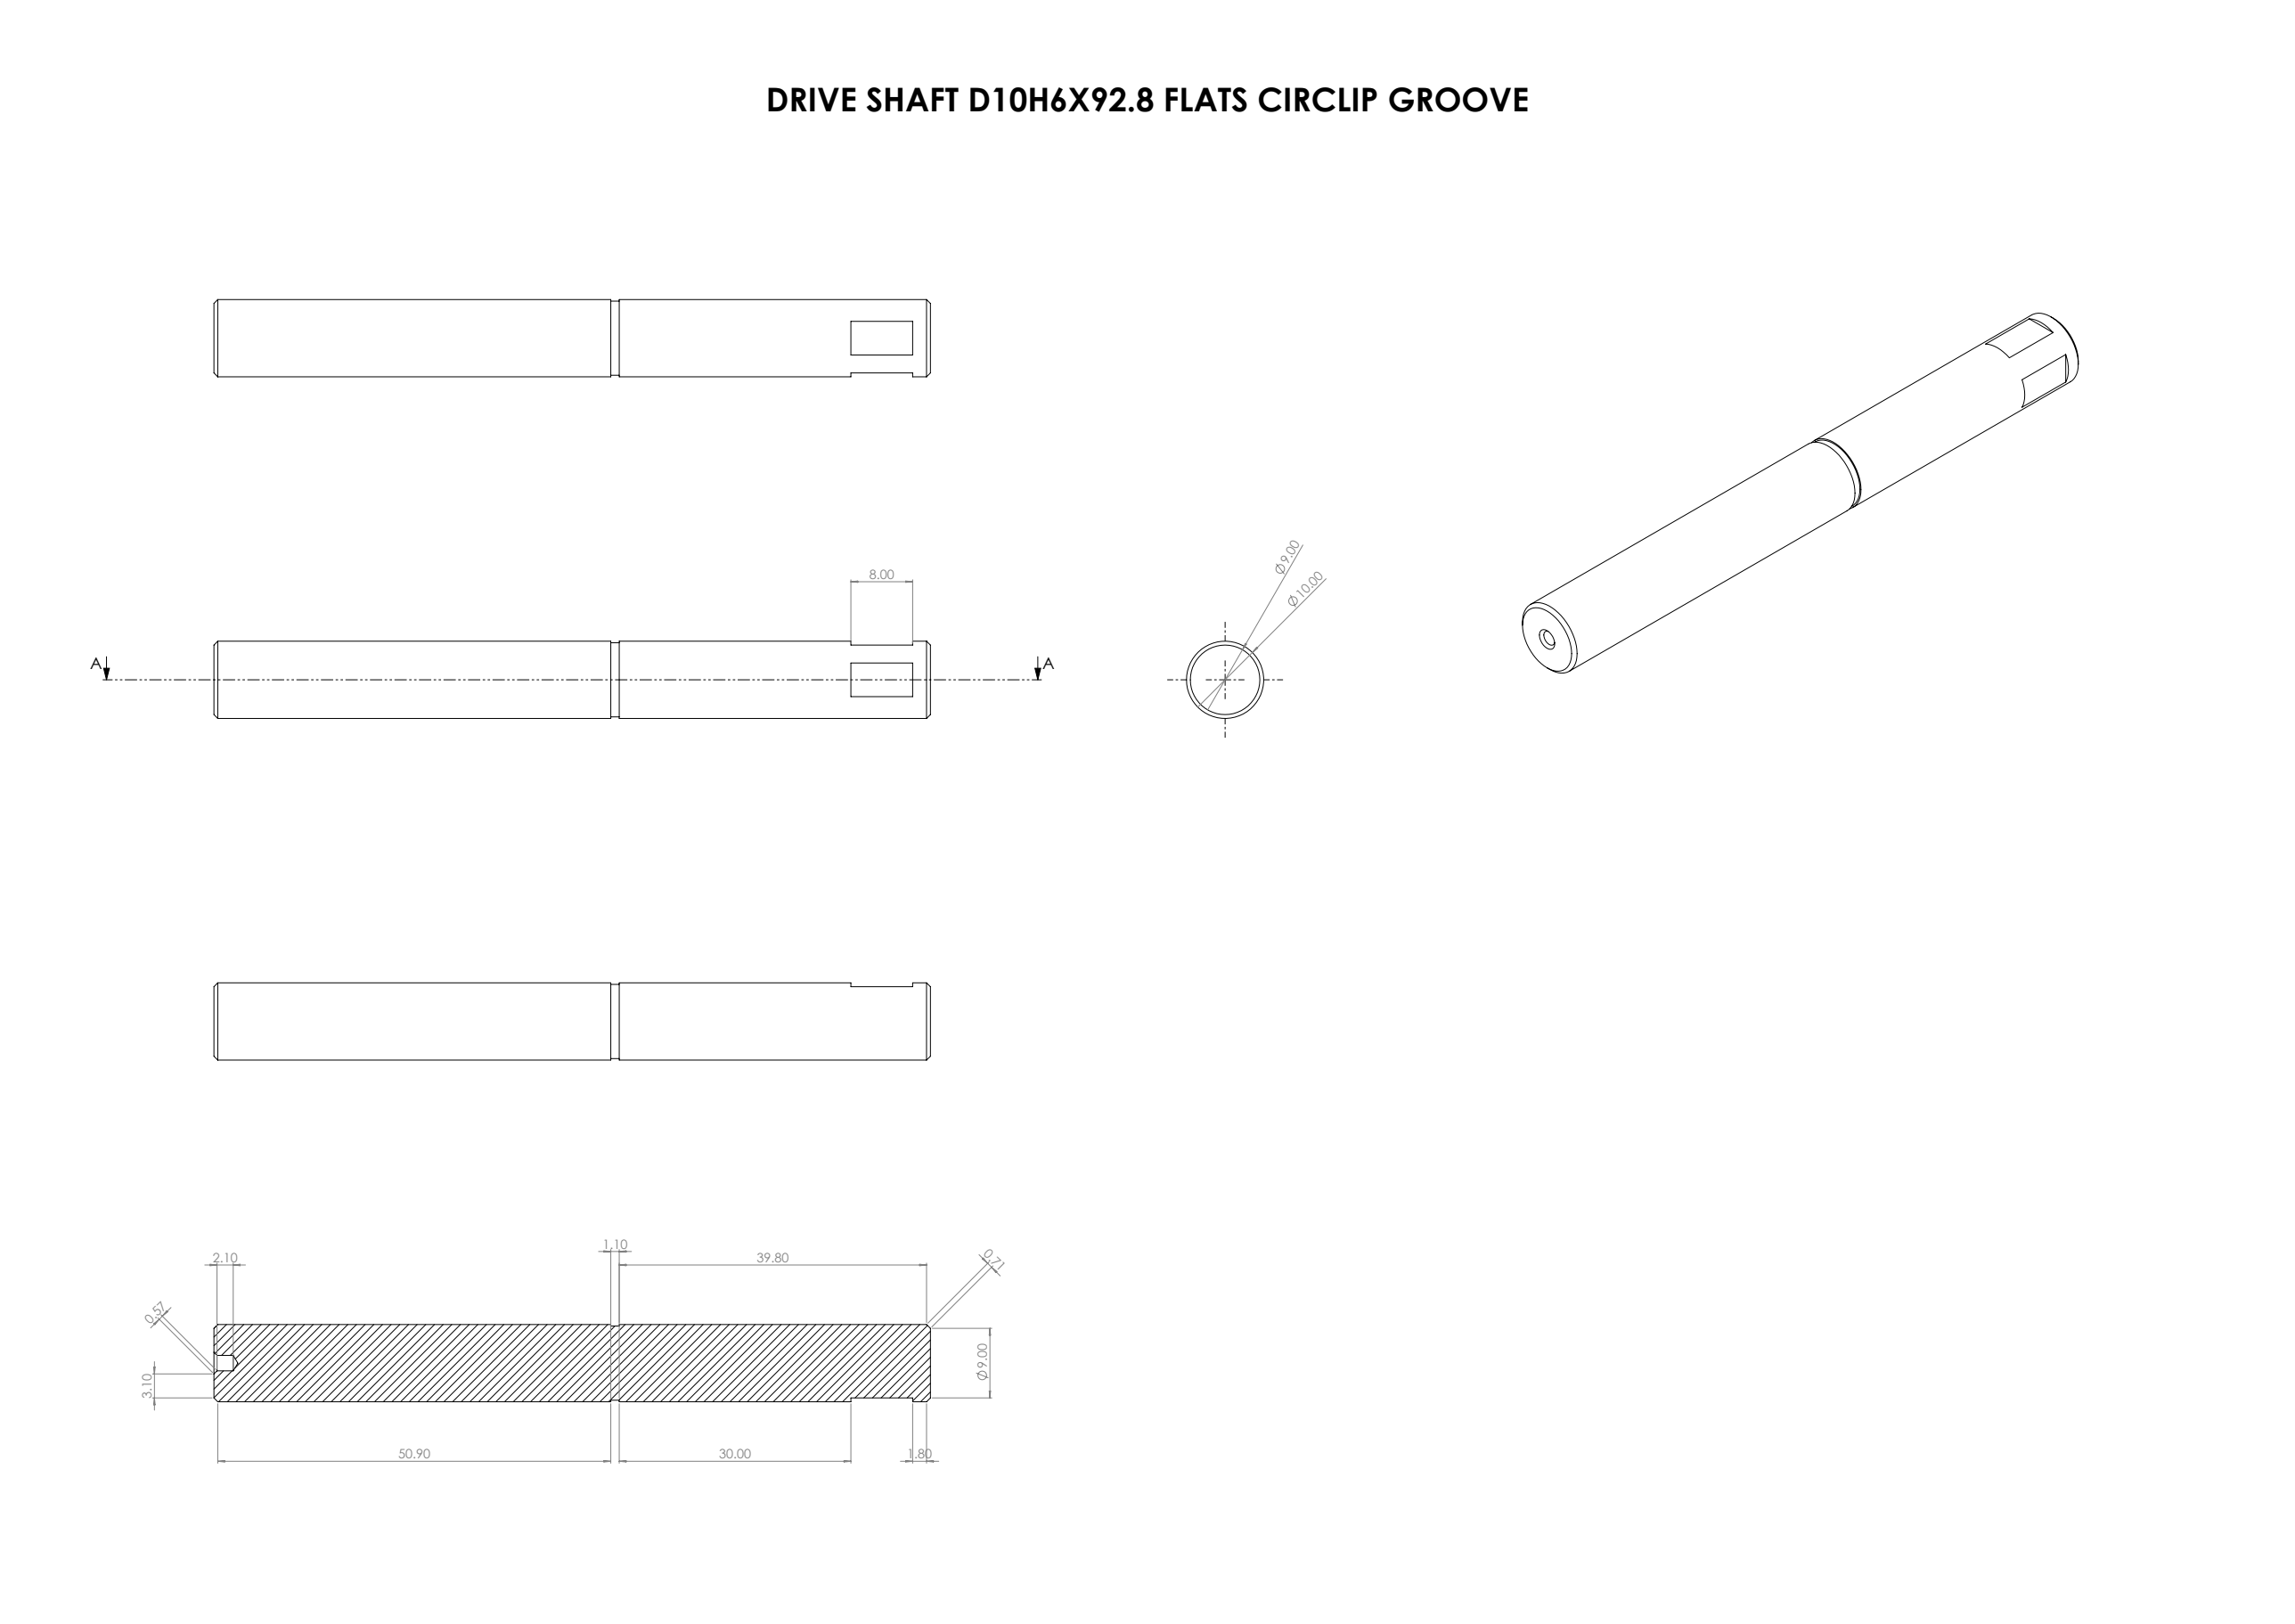
ISO-10303-21;
HEADER;
/* Generated by software containing ST-Developer
 * from STEP Tools, Inc. (www.steptools.com) 
 */

FILE_DESCRIPTION(
/* description */ (''),
/* implementation_level */ '2;1');

FILE_NAME(
/* name */ 
'02_Drive_Shaft_D10h6x92.8_Flats_Circlip_Groove.step',
/* time_stamp */ '2026-10-22T00:21:42-07:00',
/* author */ (''),
/* organization */ (''),
/* preprocessor_version */ 'ST-DEVELOPER v20.2',
/* originating_system */ 'Autodesk Translation Framework v15.15.0.0',
/* authorisation */ '');

FILE_SCHEMA (('AUTOMOTIVE_DESIGN { 1 0 10303 214 3 1 1 }'));
ENDSEC;

DATA;
#10=MECHANICAL_DESIGN_GEOMETRIC_PRESENTATION_REPRESENTATION('',(#207),#31638);
#185=SHAPE_REPRESENTATION_RELATIONSHIP('SRR','None',#31707,#196);
#196=ADVANCED_BREP_SHAPE_REPRESENTATION('',(#218),#31629);
#207=STYLED_ITEM('',(#31830),#218);
#218=MANIFOLD_SOLID_BREP('Shaft',#12482);
#268=CYLINDRICAL_SURFACE('',#12870,0.1);
#269=CYLINDRICAL_SURFACE('',#12889,0.5);
#270=CYLINDRICAL_SURFACE('',#12893,0.48);
#271=CYLINDRICAL_SURFACE('',#12897,0.5);
#402=CONICAL_SURFACE('',#12866,0.12,0.785398163397459);
#403=CONICAL_SURFACE('',#12874,0.05,1.03037682652432);
#404=CONICAL_SURFACE('',#12887,0.475,0.785398163397448);
#405=CONICAL_SURFACE('',#12899,0.475,0.785398163397441);
#1365=FACE_BOUND('',#2766,.T.);
#1366=FACE_BOUND('',#2777,.T.);
#1367=FACE_BOUND('',#2778,.T.);
#1368=FACE_BOUND('',#2780,.T.);
#1369=FACE_BOUND('',#2783,.T.);
#1511=CIRCLE('',#12867,0.14);
#1512=CIRCLE('',#12868,0.1);
#1513=CIRCLE('',#12869,0.1);
#1514=CIRCLE('',#12871,0.1);
#1515=CIRCLE('',#12873,0.45);
#1516=CIRCLE('',#12876,0.5);
#1517=CIRCLE('',#12878,0.5);
#1518=CIRCLE('',#12881,0.5);
#1519=CIRCLE('',#12884,0.5);
#1520=CIRCLE('',#12886,0.45);
#1521=CIRCLE('',#12888,0.5);
#1522=CIRCLE('',#12890,0.5);
#1523=CIRCLE('',#12892,0.48);
#1524=CIRCLE('',#12894,0.48);
#1525=CIRCLE('',#12896,0.5);
#1526=CIRCLE('',#12898,0.5);
#2044=FACE_OUTER_BOUND('',#2763,.T.);
#2045=FACE_OUTER_BOUND('',#2764,.T.);
#2046=FACE_OUTER_BOUND('',#2765,.T.);
#2047=FACE_OUTER_BOUND('',#2767,.T.);
#2048=FACE_OUTER_BOUND('',#2768,.T.);
#2049=FACE_OUTER_BOUND('',#2769,.T.);
#2050=FACE_OUTER_BOUND('',#2770,.T.);
#2051=FACE_OUTER_BOUND('',#2771,.T.);
#2052=FACE_OUTER_BOUND('',#2772,.T.);
#2053=FACE_OUTER_BOUND('',#2773,.T.);
#2054=FACE_OUTER_BOUND('',#2774,.T.);
#2055=FACE_OUTER_BOUND('',#2775,.T.);
#2056=FACE_OUTER_BOUND('',#2776,.T.);
#2057=FACE_OUTER_BOUND('',#2779,.T.);
#2058=FACE_OUTER_BOUND('',#2781,.T.);
#2059=FACE_OUTER_BOUND('',#2782,.T.);
#2060=FACE_OUTER_BOUND('',#2784,.T.);
#2061=FACE_OUTER_BOUND('',#2785,.T.);
#2763=EDGE_LOOP('',(#8981,#8982,#8983,#8984,#8985));
#2764=EDGE_LOOP('',(#8986,#8987,#8988,#8989,#8990));
#2765=EDGE_LOOP('',(#8991));
#2766=EDGE_LOOP('',(#8992));
#2767=EDGE_LOOP('',(#8993,#8994,#8995));
#2768=EDGE_LOOP('',(#8996,#8997));
#2769=EDGE_LOOP('',(#8998,#8999));
#2770=EDGE_LOOP('',(#9000,#9001,#9002,#9003));
#2771=EDGE_LOOP('',(#9004,#9005));
#2772=EDGE_LOOP('',(#9006,#9007,#9008,#9009));
#2773=EDGE_LOOP('',(#9010,#9011));
#2774=EDGE_LOOP('',(#9012));
#2775=EDGE_LOOP('',(#9013,#9014,#9015,#9016));
#2776=EDGE_LOOP('',(#9017,#9018,#9019,#9020));
#2777=EDGE_LOOP('',(#9021,#9022,#9023,#9024));
#2778=EDGE_LOOP('',(#9025,#9026,#9027,#9028));
#2779=EDGE_LOOP('',(#9029));
#2780=EDGE_LOOP('',(#9030));
#2781=EDGE_LOOP('',(#9031,#9032,#9033,#9034));
#2782=EDGE_LOOP('',(#9035));
#2783=EDGE_LOOP('',(#9036));
#2784=EDGE_LOOP('',(#9037,#9038,#9039,#9040));
#2785=EDGE_LOOP('',(#9041,#9042,#9043,#9044));
#3514=LINE('',#21084,#4219);
#3515=LINE('',#21091,#4220);
#3516=LINE('',#21097,#4221);
#3517=LINE('',#21102,#4222);
#3518=LINE('',#21107,#4223);
#3519=LINE('',#21109,#4224);
#3520=LINE('',#21110,#4225);
#3521=LINE('',#21115,#4226);
#3522=LINE('',#21118,#4227);
#3523=LINE('',#21120,#4228);
#3524=LINE('',#21121,#4229);
#3525=LINE('',#21130,#4230);
#3526=LINE('',#21134,#4231);
#3527=LINE('',#21141,#4232);
#3528=LINE('',#21148,#4233);
#3529=LINE('',#21150,#4234);
#4219=VECTOR('',#14372,0.12);
#4220=VECTOR('',#14381,0.1);
#4221=VECTOR('',#14388,0.05);
#4222=VECTOR('',#14393,1.);
#4223=VECTOR('',#14398,1.);
#4224=VECTOR('',#14401,1.);
#4225=VECTOR('',#14402,1.);
#4226=VECTOR('',#14407,1.);
#4227=VECTOR('',#14410,1.);
#4228=VECTOR('',#14411,1.);
#4229=VECTOR('',#14412,1.);
#4230=VECTOR('',#14425,0.475);
#4231=VECTOR('',#14430,0.5);
#4232=VECTOR('',#14439,0.48);
#4233=VECTOR('',#14448,0.5);
#4234=VECTOR('',#14451,0.475);
#5080=VERTEX_POINT('',#21081);
#5081=VERTEX_POINT('',#21083);
#5082=VERTEX_POINT('',#21085);
#5083=VERTEX_POINT('',#21089);
#5084=VERTEX_POINT('',#21093);
#5085=VERTEX_POINT('',#21096);
#5086=VERTEX_POINT('',#21099);
#5087=VERTEX_POINT('',#21100);
#5088=VERTEX_POINT('',#21104);
#5089=VERTEX_POINT('',#21105);
#5090=VERTEX_POINT('',#21112);
#5091=VERTEX_POINT('',#21113);
#5092=VERTEX_POINT('',#21117);
#5093=VERTEX_POINT('',#21119);
#5094=VERTEX_POINT('',#21125);
#5095=VERTEX_POINT('',#21128);
#5096=VERTEX_POINT('',#21132);
#5097=VERTEX_POINT('',#21136);
#5098=VERTEX_POINT('',#21139);
#5099=VERTEX_POINT('',#21143);
#5100=VERTEX_POINT('',#21146);
#6502=EDGE_CURVE('',#5080,#5080,#1511,.T.);
#6503=EDGE_CURVE('',#5080,#5081,#3514,.T.);
#6504=EDGE_CURVE('',#5081,#5082,#1512,.T.);
#6505=EDGE_CURVE('',#5082,#5081,#1513,.T.);
#6506=EDGE_CURVE('',#5083,#5083,#1514,.T.);
#6507=EDGE_CURVE('',#5083,#5082,#3515,.T.);
#6508=EDGE_CURVE('',#5084,#5084,#1515,.T.);
#6509=EDGE_CURVE('',#5085,#5083,#3516,.T.);
#6510=EDGE_CURVE('',#5086,#5087,#1516,.T.);
#6511=EDGE_CURVE('',#5086,#5087,#3517,.T.);
#6512=EDGE_CURVE('',#5088,#5089,#1517,.T.);
#6513=EDGE_CURVE('',#5088,#5089,#3518,.T.);
#6514=EDGE_CURVE('',#5089,#5086,#3519,.T.);
#6515=EDGE_CURVE('',#5087,#5088,#3520,.T.);
#6516=EDGE_CURVE('',#5090,#5091,#1518,.T.);
#6517=EDGE_CURVE('',#5091,#5090,#3521,.T.);
#6518=EDGE_CURVE('',#5092,#5090,#3522,.T.);
#6519=EDGE_CURVE('',#5092,#5093,#3523,.T.);
#6520=EDGE_CURVE('',#5091,#5093,#3524,.T.);
#6521=EDGE_CURVE('',#5093,#5092,#1519,.T.);
#6522=EDGE_CURVE('',#5094,#5094,#1520,.T.);
#6523=EDGE_CURVE('',#5095,#5095,#1521,.T.);
#6524=EDGE_CURVE('',#5095,#5094,#3525,.T.);
#6525=EDGE_CURVE('',#5096,#5096,#1522,.T.);
#6526=EDGE_CURVE('',#5096,#5095,#3526,.T.);
#6527=EDGE_CURVE('',#5097,#5097,#1523,.T.);
#6528=EDGE_CURVE('',#5098,#5098,#1524,.T.);
#6529=EDGE_CURVE('',#5098,#5097,#3527,.T.);
#6530=EDGE_CURVE('',#5099,#5099,#1525,.T.);
#6531=EDGE_CURVE('',#5100,#5100,#1526,.T.);
#6532=EDGE_CURVE('',#5100,#5099,#3528,.T.);
#6533=EDGE_CURVE('',#5084,#5100,#3529,.T.);
#8981=ORIENTED_EDGE('',*,*,#6502,.T.);
#8982=ORIENTED_EDGE('',*,*,#6503,.T.);
#8983=ORIENTED_EDGE('',*,*,#6504,.T.);
#8984=ORIENTED_EDGE('',*,*,#6505,.T.);
#8985=ORIENTED_EDGE('',*,*,#6503,.F.);
#8986=ORIENTED_EDGE('',*,*,#6506,.F.);
#8987=ORIENTED_EDGE('',*,*,#6507,.T.);
#8988=ORIENTED_EDGE('',*,*,#6504,.F.);
#8989=ORIENTED_EDGE('',*,*,#6505,.F.);
#8990=ORIENTED_EDGE('',*,*,#6507,.F.);
#8991=ORIENTED_EDGE('',*,*,#6508,.T.);
#8992=ORIENTED_EDGE('',*,*,#6502,.F.);
#8993=ORIENTED_EDGE('',*,*,#6509,.T.);
#8994=ORIENTED_EDGE('',*,*,#6506,.T.);
#8995=ORIENTED_EDGE('',*,*,#6509,.F.);
#8996=ORIENTED_EDGE('',*,*,#6510,.F.);
#8997=ORIENTED_EDGE('',*,*,#6511,.T.);
#8998=ORIENTED_EDGE('',*,*,#6512,.F.);
#8999=ORIENTED_EDGE('',*,*,#6513,.T.);
#9000=ORIENTED_EDGE('',*,*,#6514,.F.);
#9001=ORIENTED_EDGE('',*,*,#6513,.F.);
#9002=ORIENTED_EDGE('',*,*,#6515,.F.);
#9003=ORIENTED_EDGE('',*,*,#6511,.F.);
#9004=ORIENTED_EDGE('',*,*,#6516,.F.);
#9005=ORIENTED_EDGE('',*,*,#6517,.F.);
#9006=ORIENTED_EDGE('',*,*,#6518,.F.);
#9007=ORIENTED_EDGE('',*,*,#6519,.T.);
#9008=ORIENTED_EDGE('',*,*,#6520,.F.);
#9009=ORIENTED_EDGE('',*,*,#6517,.T.);
#9010=ORIENTED_EDGE('',*,*,#6521,.F.);
#9011=ORIENTED_EDGE('',*,*,#6519,.F.);
#9012=ORIENTED_EDGE('',*,*,#6522,.F.);
#9013=ORIENTED_EDGE('',*,*,#6523,.F.);
#9014=ORIENTED_EDGE('',*,*,#6524,.T.);
#9015=ORIENTED_EDGE('',*,*,#6522,.T.);
#9016=ORIENTED_EDGE('',*,*,#6524,.F.);
#9017=ORIENTED_EDGE('',*,*,#6525,.F.);
#9018=ORIENTED_EDGE('',*,*,#6526,.T.);
#9019=ORIENTED_EDGE('',*,*,#6523,.T.);
#9020=ORIENTED_EDGE('',*,*,#6526,.F.);
#9021=ORIENTED_EDGE('',*,*,#6512,.T.);
#9022=ORIENTED_EDGE('',*,*,#6514,.T.);
#9023=ORIENTED_EDGE('',*,*,#6510,.T.);
#9024=ORIENTED_EDGE('',*,*,#6515,.T.);
#9025=ORIENTED_EDGE('',*,*,#6520,.T.);
#9026=ORIENTED_EDGE('',*,*,#6521,.T.);
#9027=ORIENTED_EDGE('',*,*,#6518,.T.);
#9028=ORIENTED_EDGE('',*,*,#6516,.T.);
#9029=ORIENTED_EDGE('',*,*,#6525,.T.);
#9030=ORIENTED_EDGE('',*,*,#6527,.F.);
#9031=ORIENTED_EDGE('',*,*,#6528,.F.);
#9032=ORIENTED_EDGE('',*,*,#6529,.T.);
#9033=ORIENTED_EDGE('',*,*,#6527,.T.);
#9034=ORIENTED_EDGE('',*,*,#6529,.F.);
#9035=ORIENTED_EDGE('',*,*,#6530,.F.);
#9036=ORIENTED_EDGE('',*,*,#6528,.T.);
#9037=ORIENTED_EDGE('',*,*,#6531,.F.);
#9038=ORIENTED_EDGE('',*,*,#6532,.T.);
#9039=ORIENTED_EDGE('',*,*,#6530,.T.);
#9040=ORIENTED_EDGE('',*,*,#6532,.F.);
#9041=ORIENTED_EDGE('',*,*,#6508,.F.);
#9042=ORIENTED_EDGE('',*,*,#6533,.T.);
#9043=ORIENTED_EDGE('',*,*,#6531,.T.);
#9044=ORIENTED_EDGE('',*,*,#6533,.F.);
#11560=PLANE('',#12872);
#11561=PLANE('',#12875);
#11562=PLANE('',#12877);
#11563=PLANE('',#12879);
#11564=PLANE('',#12880);
#11565=PLANE('',#12882);
#11566=PLANE('',#12883);
#11567=PLANE('',#12885);
#11568=PLANE('',#12891);
#11569=PLANE('',#12895);
#12011=ADVANCED_FACE('',(#2044),#402,.F.);
#12012=ADVANCED_FACE('',(#2045),#268,.F.);
#12013=ADVANCED_FACE('',(#2046,#1365),#11560,.T.);
#12014=ADVANCED_FACE('',(#2047),#403,.F.);
#12015=ADVANCED_FACE('',(#2048),#11561,.F.);
#12016=ADVANCED_FACE('',(#2049),#11562,.F.);
#12017=ADVANCED_FACE('',(#2050),#11563,.F.);
#12018=ADVANCED_FACE('',(#2051),#11564,.F.);
#12019=ADVANCED_FACE('',(#2052),#11565,.F.);
#12020=ADVANCED_FACE('',(#2053),#11566,.F.);
#12021=ADVANCED_FACE('',(#2054),#11567,.T.);
#12022=ADVANCED_FACE('',(#2055),#404,.T.);
#12023=ADVANCED_FACE('',(#2056,#1366,#1367),#269,.T.);
#12024=ADVANCED_FACE('',(#2057,#1368),#11568,.T.);
#12025=ADVANCED_FACE('',(#2058),#270,.T.);
#12026=ADVANCED_FACE('',(#2059,#1369),#11569,.T.);
#12027=ADVANCED_FACE('',(#2060),#271,.T.);
#12028=ADVANCED_FACE('',(#2061),#405,.T.);
#12482=CLOSED_SHELL('',(#12011,#12012,#12013,#12014,#12015,#12016,#12017,
#12018,#12019,#12020,#12021,#12022,#12023,#12024,#12025,#12026,#12027,#12028));
#12865=AXIS2_PLACEMENT_3D('',#21079,#14366,#14367);
#12866=AXIS2_PLACEMENT_3D('',#21080,#14368,#14369);
#12867=AXIS2_PLACEMENT_3D('',#21082,#14370,#14371);
#12868=AXIS2_PLACEMENT_3D('',#21086,#14373,#14374);
#12869=AXIS2_PLACEMENT_3D('',#21087,#14375,#14376);
#12870=AXIS2_PLACEMENT_3D('',#21088,#14377,#14378);
#12871=AXIS2_PLACEMENT_3D('',#21090,#14379,#14380);
#12872=AXIS2_PLACEMENT_3D('',#21092,#14382,#14383);
#12873=AXIS2_PLACEMENT_3D('',#21094,#14384,#14385);
#12874=AXIS2_PLACEMENT_3D('',#21095,#14386,#14387);
#12875=AXIS2_PLACEMENT_3D('',#21098,#14389,#14390);
#12876=AXIS2_PLACEMENT_3D('',#21101,#14391,#14392);
#12877=AXIS2_PLACEMENT_3D('',#21103,#14394,#14395);
#12878=AXIS2_PLACEMENT_3D('',#21106,#14396,#14397);
#12879=AXIS2_PLACEMENT_3D('',#21108,#14399,#14400);
#12880=AXIS2_PLACEMENT_3D('',#21111,#14403,#14404);
#12881=AXIS2_PLACEMENT_3D('',#21114,#14405,#14406);
#12882=AXIS2_PLACEMENT_3D('',#21116,#14408,#14409);
#12883=AXIS2_PLACEMENT_3D('',#21122,#14413,#14414);
#12884=AXIS2_PLACEMENT_3D('',#21123,#14415,#14416);
#12885=AXIS2_PLACEMENT_3D('',#21124,#14417,#14418);
#12886=AXIS2_PLACEMENT_3D('',#21126,#14419,#14420);
#12887=AXIS2_PLACEMENT_3D('',#21127,#14421,#14422);
#12888=AXIS2_PLACEMENT_3D('',#21129,#14423,#14424);
#12889=AXIS2_PLACEMENT_3D('',#21131,#14426,#14427);
#12890=AXIS2_PLACEMENT_3D('',#21133,#14428,#14429);
#12891=AXIS2_PLACEMENT_3D('',#21135,#14431,#14432);
#12892=AXIS2_PLACEMENT_3D('',#21137,#14433,#14434);
#12893=AXIS2_PLACEMENT_3D('',#21138,#14435,#14436);
#12894=AXIS2_PLACEMENT_3D('',#21140,#14437,#14438);
#12895=AXIS2_PLACEMENT_3D('',#21142,#14440,#14441);
#12896=AXIS2_PLACEMENT_3D('',#21144,#14442,#14443);
#12897=AXIS2_PLACEMENT_3D('',#21145,#14444,#14445);
#12898=AXIS2_PLACEMENT_3D('',#21147,#14446,#14447);
#12899=AXIS2_PLACEMENT_3D('',#21149,#14449,#14450);
#14366=DIRECTION('axis',(0.,0.,1.));
#14367=DIRECTION('refdir',(1.,0.,0.));
#14368=DIRECTION('center_axis',(0.,0.,1.));
#14369=DIRECTION('ref_axis',(-1.,0.,0.));
#14370=DIRECTION('center_axis',(0.,0.,1.));
#14371=DIRECTION('ref_axis',(-1.,0.,0.));
#14372=DIRECTION('',(-0.707106781186555,-8.65956056235503E-17,-0.70710678118654));
#14373=DIRECTION('center_axis',(0.,0.,-1.));
#14374=DIRECTION('ref_axis',(-1.,0.,0.));
#14375=DIRECTION('center_axis',(0.,0.,-1.));
#14376=DIRECTION('ref_axis',(-1.,0.,0.));
#14377=DIRECTION('center_axis',(0.,0.,1.));
#14378=DIRECTION('ref_axis',(1.,0.,0.));
#14379=DIRECTION('center_axis',(0.,0.,1.));
#14380=DIRECTION('ref_axis',(1.,0.,0.));
#14381=DIRECTION('',(0.,0.,1.));
#14382=DIRECTION('center_axis',(0.,0.,1.));
#14383=DIRECTION('ref_axis',(1.,0.,0.));
#14384=DIRECTION('center_axis',(0.,0.,1.));
#14385=DIRECTION('ref_axis',(1.,0.,0.));
#14386=DIRECTION('center_axis',(0.,0.,1.));
#14387=DIRECTION('ref_axis',(1.,0.,0.));
#14388=DIRECTION('',(-0.857492925712549,-1.05012596676537E-16,0.514495755427518));
#14389=DIRECTION('center_axis',(0.,0.,1.));
#14390=DIRECTION('ref_axis',(0.,-1.,0.));
#14391=DIRECTION('center_axis',(0.,0.,1.));
#14392=DIRECTION('ref_axis',(1.,0.,0.));
#14393=DIRECTION('',(-1.,0.,0.));
#14394=DIRECTION('center_axis',(0.,0.,-1.));
#14395=DIRECTION('ref_axis',(0.,1.,0.));
#14396=DIRECTION('center_axis',(0.,0.,-1.));
#14397=DIRECTION('ref_axis',(1.,0.,0.));
#14398=DIRECTION('',(1.,0.,0.));
#14399=DIRECTION('center_axis',(0.,-1.,0.));
#14400=DIRECTION('ref_axis',(0.,0.,-1.));
#14401=DIRECTION('',(0.,0.,1.));
#14402=DIRECTION('',(0.,0.,-1.));
#14403=DIRECTION('center_axis',(0.,0.,-1.));
#14404=DIRECTION('ref_axis',(-1.,0.,0.));
#14405=DIRECTION('center_axis',(0.,0.,-1.));
#14406=DIRECTION('ref_axis',(1.,0.,0.));
#14407=DIRECTION('',(0.,1.,0.));
#14408=DIRECTION('center_axis',(-1.,0.,0.));
#14409=DIRECTION('ref_axis',(0.,0.,1.));
#14410=DIRECTION('',(0.,0.,-1.));
#14411=DIRECTION('',(0.,-1.,0.));
#14412=DIRECTION('',(0.,0.,1.));
#14413=DIRECTION('center_axis',(0.,0.,1.));
#14414=DIRECTION('ref_axis',(1.,0.,0.));
#14415=DIRECTION('center_axis',(0.,0.,1.));
#14416=DIRECTION('ref_axis',(1.,0.,0.));
#14417=DIRECTION('center_axis',(0.,0.,-1.));
#14418=DIRECTION('ref_axis',(-1.,0.,0.));
#14419=DIRECTION('center_axis',(0.,0.,1.));
#14420=DIRECTION('ref_axis',(1.,0.,0.));
#14421=DIRECTION('center_axis',(0.,0.,1.));
#14422=DIRECTION('ref_axis',(1.,0.,0.));
#14423=DIRECTION('center_axis',(0.,0.,1.));
#14424=DIRECTION('ref_axis',(1.,0.,0.));
#14425=DIRECTION('',(0.707106781186547,8.65956056235493E-17,-0.707106781186548));
#14426=DIRECTION('center_axis',(0.,0.,1.));
#14427=DIRECTION('ref_axis',(1.,0.,0.));
#14428=DIRECTION('center_axis',(0.,0.,1.));
#14429=DIRECTION('ref_axis',(1.,0.,0.));
#14430=DIRECTION('',(0.,0.,-1.));
#14431=DIRECTION('center_axis',(0.,0.,1.));
#14432=DIRECTION('ref_axis',(1.,0.,0.));
#14433=DIRECTION('center_axis',(0.,0.,1.));
#14434=DIRECTION('ref_axis',(1.,0.,0.));
#14435=DIRECTION('center_axis',(0.,0.,1.));
#14436=DIRECTION('ref_axis',(1.,0.,0.));
#14437=DIRECTION('center_axis',(0.,0.,1.));
#14438=DIRECTION('ref_axis',(1.,0.,0.));
#14439=DIRECTION('',(0.,0.,-1.));
#14440=DIRECTION('center_axis',(0.,0.,-1.));
#14441=DIRECTION('ref_axis',(-1.,0.,0.));
#14442=DIRECTION('center_axis',(0.,0.,1.));
#14443=DIRECTION('ref_axis',(1.,0.,0.));
#14444=DIRECTION('center_axis',(0.,0.,1.));
#14445=DIRECTION('ref_axis',(1.,0.,0.));
#14446=DIRECTION('center_axis',(0.,0.,1.));
#14447=DIRECTION('ref_axis',(1.,0.,0.));
#14448=DIRECTION('',(0.,0.,-1.));
#14449=DIRECTION('center_axis',(0.,0.,-1.));
#14450=DIRECTION('ref_axis',(1.,0.,0.));
#14451=DIRECTION('',(-0.707106781186542,-8.65956056235487E-17,-0.707106781186553));
#21079=CARTESIAN_POINT('',(0.,0.,0.));
#21080=CARTESIAN_POINT('Origin',(0.,0.,10.98));
#21081=CARTESIAN_POINT('',(0.14,1.71450551880629E-17,11.));
#21082=CARTESIAN_POINT('Origin',(0.,0.,11.));
#21083=CARTESIAN_POINT('',(0.1,-1.22464679914735E-17,10.96));
#21084=CARTESIAN_POINT('',(0.12,1.46957615897682E-17,10.98));
#21085=CARTESIAN_POINT('',(-0.1,-1.22464679914735E-17,10.96));
#21086=CARTESIAN_POINT('Origin',(0.,0.,10.96));
#21087=CARTESIAN_POINT('Origin',(0.,0.,10.96));
#21088=CARTESIAN_POINT('Origin',(0.,0.,10.875));
#21089=CARTESIAN_POINT('',(-0.1,-1.22464679914735E-17,10.75));
#21090=CARTESIAN_POINT('Origin',(0.,0.,10.75));
#21091=CARTESIAN_POINT('',(-0.1,-1.22464679914735E-17,10.875));
#21092=CARTESIAN_POINT('Origin',(0.,0.,11.));
#21093=CARTESIAN_POINT('',(-0.45,-5.51091059616309E-17,11.));
#21094=CARTESIAN_POINT('Origin',(0.,0.,11.));
#21095=CARTESIAN_POINT('Origin',(0.,0.,10.72));
#21096=CARTESIAN_POINT('',(0.,0.,10.69));
#21097=CARTESIAN_POINT('',(-0.05,-6.12323399573677E-18,10.72));
#21098=CARTESIAN_POINT('Origin',(0.,0.6,2.75));
#21099=CARTESIAN_POINT('',(0.217944947177034,0.45,2.75));
#21100=CARTESIAN_POINT('',(-0.217944947177034,0.45,2.75));
#21101=CARTESIAN_POINT('Origin',(0.,0.,2.75));
#21102=CARTESIAN_POINT('',(0.,0.45,2.75));
#21103=CARTESIAN_POINT('Origin',(0.,0.45,1.95));
#21104=CARTESIAN_POINT('',(-0.217944947177034,0.45,1.95));
#21105=CARTESIAN_POINT('',(0.217944947177034,0.45,1.95));
#21106=CARTESIAN_POINT('Origin',(0.,0.,1.95));
#21107=CARTESIAN_POINT('',(0.,0.45,1.95));
#21108=CARTESIAN_POINT('Origin',(0.,0.45,2.75));
#21109=CARTESIAN_POINT('',(0.217944947177034,0.45,3.76));
#21110=CARTESIAN_POINT('',(-0.217944947177034,0.45,3.76));
#21111=CARTESIAN_POINT('Origin',(0.6,0.,1.95));
#21112=CARTESIAN_POINT('',(0.45,0.217944947177034,1.95));
#21113=CARTESIAN_POINT('',(0.45,-0.217944947177034,1.95));
#21114=CARTESIAN_POINT('Origin',(0.,0.,1.95));
#21115=CARTESIAN_POINT('',(0.45,0.,1.95));
#21116=CARTESIAN_POINT('Origin',(0.45,0.,1.95));
#21117=CARTESIAN_POINT('',(0.45,0.217944947177034,2.75));
#21118=CARTESIAN_POINT('',(0.45,0.217944947177034,3.76));
#21119=CARTESIAN_POINT('',(0.45,-0.217944947177034,2.75));
#21120=CARTESIAN_POINT('',(0.45,0.,2.75));
#21121=CARTESIAN_POINT('',(0.45,-0.217944947177034,3.76));
#21122=CARTESIAN_POINT('Origin',(0.45,0.,2.75));
#21123=CARTESIAN_POINT('Origin',(0.,0.,2.75));
#21124=CARTESIAN_POINT('Origin',(0.45,0.,1.72));
#21125=CARTESIAN_POINT('',(-0.45,-5.51091059616309E-17,1.72));
#21126=CARTESIAN_POINT('Origin',(0.,0.,1.72));
#21127=CARTESIAN_POINT('Origin',(0.,0.,1.745));
#21128=CARTESIAN_POINT('',(-0.499999999999999,-6.12323399573676E-17,1.77));
#21129=CARTESIAN_POINT('Origin',(0.,0.,1.77));
#21130=CARTESIAN_POINT('',(-0.475,-5.81707229594993E-17,1.745));
#21131=CARTESIAN_POINT('Origin',(0.,0.,3.76));
#21132=CARTESIAN_POINT('',(-0.5,-6.12323399573677E-17,5.75));
#21133=CARTESIAN_POINT('Origin',(0.,0.,5.75));
#21134=CARTESIAN_POINT('',(-0.5,-6.12323399573677E-17,3.76));
#21135=CARTESIAN_POINT('Origin',(0.48,0.,5.75));
#21136=CARTESIAN_POINT('',(-0.48,-5.87830463590729E-17,5.75));
#21137=CARTESIAN_POINT('Origin',(0.,0.,5.75));
#21138=CARTESIAN_POINT('Origin',(0.,0.,5.805));
#21139=CARTESIAN_POINT('',(-0.48,-5.87830463590729E-17,5.86));
#21140=CARTESIAN_POINT('Origin',(0.,0.,5.86));
#21141=CARTESIAN_POINT('',(-0.48,-5.87830463590729E-17,5.805));
#21142=CARTESIAN_POINT('Origin',(0.5,0.,5.86));
#21143=CARTESIAN_POINT('',(-0.5,-6.12323399573677E-17,5.86));
#21144=CARTESIAN_POINT('Origin',(0.,0.,5.86));
#21145=CARTESIAN_POINT('Origin',(0.,0.,8.405));
#21146=CARTESIAN_POINT('',(-0.5,-6.12323399573677E-17,10.95));
#21147=CARTESIAN_POINT('Origin',(0.,0.,10.95));
#21148=CARTESIAN_POINT('',(-0.5,-6.12323399573677E-17,8.405));
#21149=CARTESIAN_POINT('Origin',(0.,0.,10.975));
#21150=CARTESIAN_POINT('',(-0.475,-5.81707229594993E-17,10.975));
#31616=UNCERTAINTY_MEASURE_WITH_UNIT(LENGTH_MEASURE(0.001),#31639,
'DISTANCE_ACCURACY_VALUE',
'Maximum model space distance between geometric entities at asserted c
onnectivities');
#31625=UNCERTAINTY_MEASURE_WITH_UNIT(LENGTH_MEASURE(0.001),#31639,
'DISTANCE_ACCURACY_VALUE',
'Maximum model space distance between geometric entities at asserted c
onnectivities');
#31629=(
GEOMETRIC_REPRESENTATION_CONTEXT(3)
GLOBAL_UNCERTAINTY_ASSIGNED_CONTEXT((#31616))
GLOBAL_UNIT_ASSIGNED_CONTEXT((#31639,#31641,#31642))
REPRESENTATION_CONTEXT('','3D')
);
#31638=(
GEOMETRIC_REPRESENTATION_CONTEXT(3)
GLOBAL_UNCERTAINTY_ASSIGNED_CONTEXT((#31625))
GLOBAL_UNIT_ASSIGNED_CONTEXT((#31639,#31641,#31642))
REPRESENTATION_CONTEXT('','3D')
);
#31639=(
LENGTH_UNIT()
NAMED_UNIT(*)
SI_UNIT(.CENTI.,.METRE.)
);
#31641=(
NAMED_UNIT(*)
PLANE_ANGLE_UNIT()
SI_UNIT($,.RADIAN.)
);
#31642=(
NAMED_UNIT(*)
SI_UNIT($,.STERADIAN.)
SOLID_ANGLE_UNIT()
);
#31646=SHAPE_DEFINITION_REPRESENTATION(#31658,#31707);
#31658=PRODUCT_DEFINITION_SHAPE('',$,#31720);
#31707=SHAPE_REPRESENTATION('',(#12865),#31629);
#31716=PRODUCT_DEFINITION_CONTEXT('part definition',#31754,'design');
#31720=PRODUCT_DEFINITION('2026-10-22-02-42-12-024',
'02_Drive_Shaft_D10h6x92.8_Flats_Circlip_Groove',#31732,#31716);
#31732=PRODUCT_DEFINITION_FORMATION('',$,#31759);
#31754=APPLICATION_CONTEXT(
'Core Data for Automotive Mechanical Design Process');
#31755=PRODUCT_CONTEXT('part definition',#31754,'mechanical');
#31759=PRODUCT('2026-10-22-02-42-12-024',
'02_Drive_Shaft_D10h6x92.8_Flats_Circlip_Groove',$,(#31755));
#31824=COLOUR_RGB('Grey',0.48,0.52,0.57);
#31825=FILL_AREA_STYLE_COLOUR('',#31824);
#31826=FILL_AREA_STYLE('',(#31825));
#31827=SURFACE_STYLE_FILL_AREA(#31826);
#31828=SURFACE_SIDE_STYLE('',(#31827));
#31829=SURFACE_STYLE_USAGE(.BOTH.,#31828);
#31830=PRESENTATION_STYLE_ASSIGNMENT((#31829));
ENDSEC;
END-ISO-10303-21;
